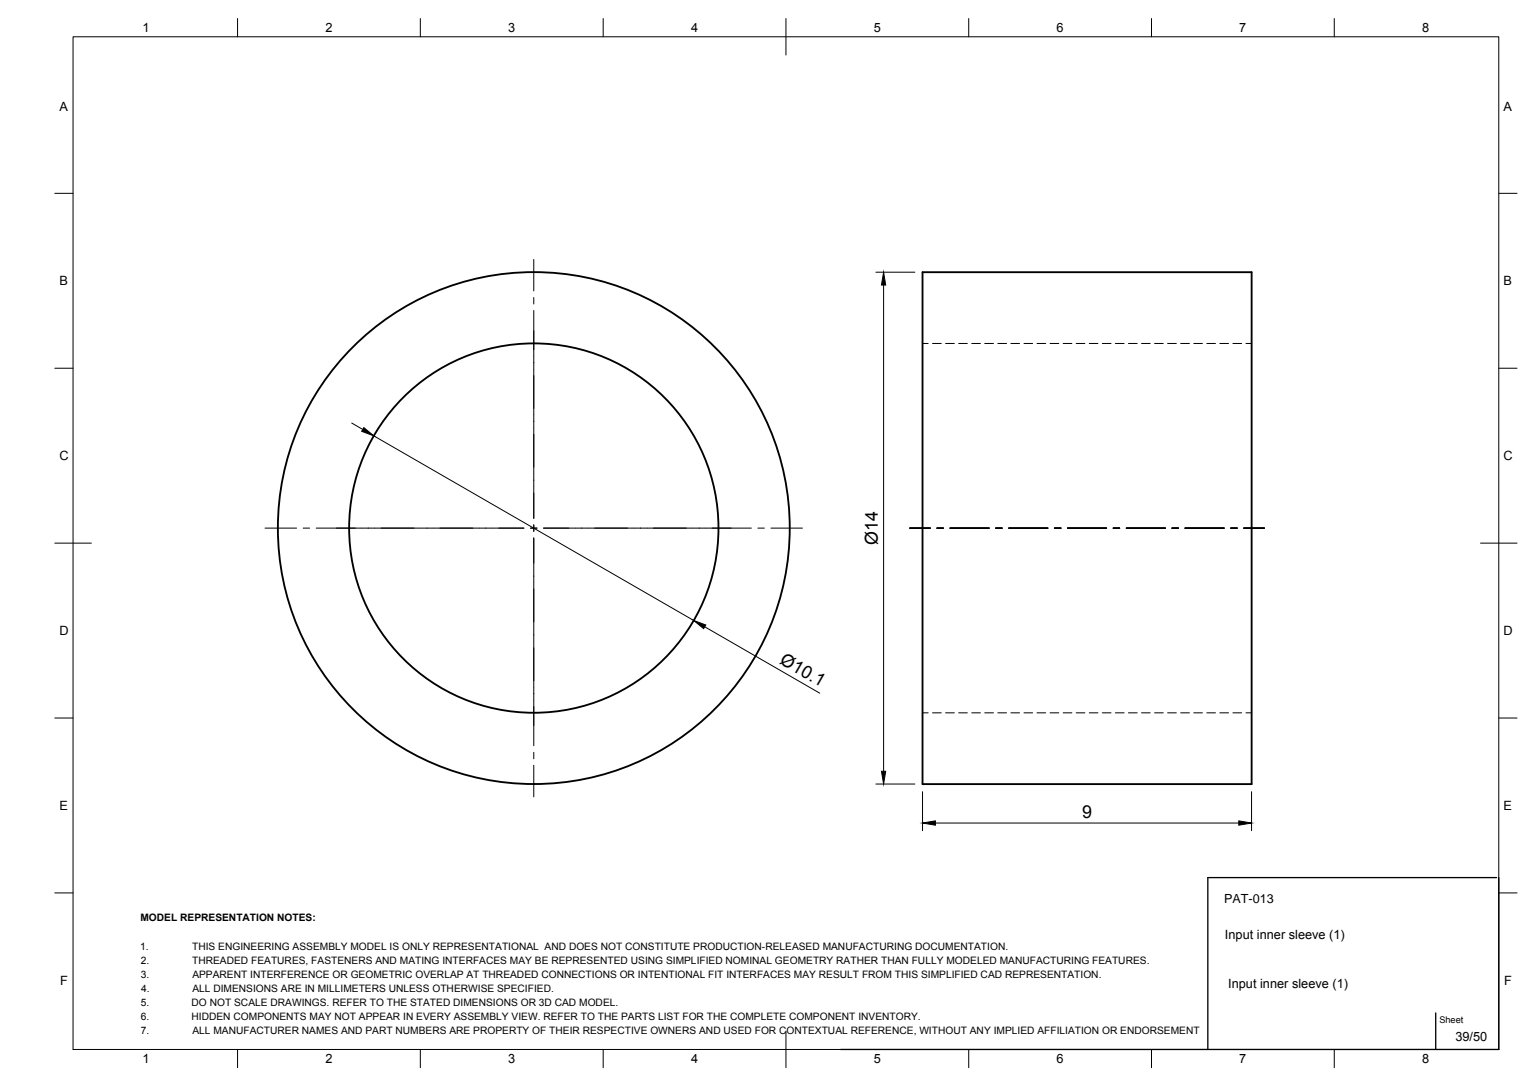
ISO-10303-21;
HEADER;
/* Generated by software containing ST-Developer
 * from STEP Tools, Inc. (www.steptools.com) 
 */

FILE_DESCRIPTION(
/* description */ ('Belt-driven linear axis on 2020 extrusion'),
/* implementation_level */ '2;1');

FILE_NAME(
/* name */ 'Input inner sleeve (1).step',
/* time_stamp */ '2026-10-28T03:26:09-07:00',
/* author */ (''),
/* organization */ (''),
/* preprocessor_version */ 'ST-DEVELOPER v20.2',
/* originating_system */ 'Autodesk Translation Framework v15.17.0.0',
/* authorisation */ '');

FILE_SCHEMA (('AUTOMOTIVE_DESIGN { 1 0 10303 214 3 1 1 }'));
ENDSEC;

DATA;
#10=MECHANICAL_DESIGN_GEOMETRIC_PRESENTATION_REPRESENTATION('',(#651),#20096);
#549=SHAPE_REPRESENTATION_RELATIONSHIP('SRR','None',#20348,#595);
#595=ADVANCED_BREP_SHAPE_REPRESENTATION('',(#706),#20079);
#651=STYLED_ITEM('',(#20636),#706);
#706=MANIFOLD_SOLID_BREP('Body1',#10965);
#847=FACE_BOUND('',#2420,.T.);
#848=FACE_BOUND('',#2422,.T.);
#1136=PLANE('',#12297);
#1137=PLANE('',#12298);
#1666=FACE_OUTER_BOUND('',#2417,.T.);
#1667=FACE_OUTER_BOUND('',#2418,.T.);
#1668=FACE_OUTER_BOUND('',#2419,.T.);
#1669=FACE_OUTER_BOUND('',#2421,.T.);
#2417=EDGE_LOOP('',(#9097,#9098,#9099,#9100));
#2418=EDGE_LOOP('',(#9101,#9102,#9103,#9104));
#2419=EDGE_LOOP('',(#9105));
#2420=EDGE_LOOP('',(#9106));
#2421=EDGE_LOOP('',(#9107));
#2422=EDGE_LOOP('',(#9108));
#3226=LINE('',#18577,#4083);
#3227=LINE('',#18583,#4084);
#4083=VECTOR('',#14952,0.505000000000003);
#4084=VECTOR('',#14959,0.700000000000003);
#4720=CIRCLE('',#12292,0.505000000000003);
#4721=CIRCLE('',#12293,0.505000000000003);
#4722=CIRCLE('',#12295,0.700000000000003);
#4723=CIRCLE('',#12296,0.700000000000003);
#5515=VERTEX_POINT('',#18574);
#5516=VERTEX_POINT('',#18576);
#5517=VERTEX_POINT('',#18580);
#5518=VERTEX_POINT('',#18582);
#6763=EDGE_CURVE('',#5515,#5515,#4720,.T.);
#6764=EDGE_CURVE('',#5515,#5516,#3226,.T.);
#6765=EDGE_CURVE('',#5516,#5516,#4721,.T.);
#6766=EDGE_CURVE('',#5517,#5517,#4722,.T.);
#6767=EDGE_CURVE('',#5517,#5518,#3227,.T.);
#6768=EDGE_CURVE('',#5518,#5518,#4723,.T.);
#9097=ORIENTED_EDGE('',*,*,#6763,.F.);
#9098=ORIENTED_EDGE('',*,*,#6764,.T.);
#9099=ORIENTED_EDGE('',*,*,#6765,.T.);
#9100=ORIENTED_EDGE('',*,*,#6764,.F.);
#9101=ORIENTED_EDGE('',*,*,#6766,.F.);
#9102=ORIENTED_EDGE('',*,*,#6767,.T.);
#9103=ORIENTED_EDGE('',*,*,#6768,.T.);
#9104=ORIENTED_EDGE('',*,*,#6767,.F.);
#9105=ORIENTED_EDGE('',*,*,#6766,.T.);
#9106=ORIENTED_EDGE('',*,*,#6763,.T.);
#9107=ORIENTED_EDGE('',*,*,#6768,.F.);
#9108=ORIENTED_EDGE('',*,*,#6765,.F.);
#10221=CYLINDRICAL_SURFACE('',#12291,0.505000000000003);
#10222=CYLINDRICAL_SURFACE('',#12294,0.700000000000003);
#10717=ADVANCED_FACE('',(#1666),#10221,.F.);
#10718=ADVANCED_FACE('',(#1667),#10222,.T.);
#10719=ADVANCED_FACE('',(#1668,#847),#1136,.T.);
#10720=ADVANCED_FACE('',(#1669,#848),#1137,.F.);
#10965=CLOSED_SHELL('',(#10717,#10718,#10719,#10720));
#12290=AXIS2_PLACEMENT_3D('',#18572,#14946,#14947);
#12291=AXIS2_PLACEMENT_3D('',#18573,#14948,#14949);
#12292=AXIS2_PLACEMENT_3D('',#18575,#14950,#14951);
#12293=AXIS2_PLACEMENT_3D('',#18578,#14953,#14954);
#12294=AXIS2_PLACEMENT_3D('',#18579,#14955,#14956);
#12295=AXIS2_PLACEMENT_3D('',#18581,#14957,#14958);
#12296=AXIS2_PLACEMENT_3D('',#18584,#14960,#14961);
#12297=AXIS2_PLACEMENT_3D('',#18585,#14962,#14963);
#12298=AXIS2_PLACEMENT_3D('',#18586,#14964,#14965);
#14946=DIRECTION('axis',(0.,0.,1.));
#14947=DIRECTION('refdir',(1.,0.,0.));
#14948=DIRECTION('center_axis',(0.,1.,0.));
#14949=DIRECTION('ref_axis',(1.,0.,0.));
#14950=DIRECTION('center_axis',(0.,-1.,0.));
#14951=DIRECTION('ref_axis',(1.,0.,0.));
#14952=DIRECTION('',(0.,-1.,0.));
#14953=DIRECTION('center_axis',(0.,-1.,0.));
#14954=DIRECTION('ref_axis',(1.,0.,0.));
#14955=DIRECTION('center_axis',(0.,1.,0.));
#14956=DIRECTION('ref_axis',(1.,0.,0.));
#14957=DIRECTION('center_axis',(0.,1.,0.));
#14958=DIRECTION('ref_axis',(1.,0.,0.));
#14959=DIRECTION('',(0.,-1.,0.));
#14960=DIRECTION('center_axis',(0.,1.,0.));
#14961=DIRECTION('ref_axis',(1.,0.,0.));
#14962=DIRECTION('center_axis',(0.,1.,0.));
#14963=DIRECTION('ref_axis',(1.,0.,0.));
#14964=DIRECTION('center_axis',(0.,1.,0.));
#14965=DIRECTION('ref_axis',(1.,0.,0.));
#18572=CARTESIAN_POINT('',(0.,0.,0.));
#18573=CARTESIAN_POINT('Origin',(32.,-0.45,7.));
#18574=CARTESIAN_POINT('',(31.495,0.45,7.));
#18575=CARTESIAN_POINT('Origin',(32.,0.45,7.));
#18576=CARTESIAN_POINT('',(31.495,-0.45,7.));
#18577=CARTESIAN_POINT('',(31.495,-0.45,7.));
#18578=CARTESIAN_POINT('Origin',(32.,-0.45,7.));
#18579=CARTESIAN_POINT('Origin',(32.,-0.45,7.));
#18580=CARTESIAN_POINT('',(31.3,0.45,7.));
#18581=CARTESIAN_POINT('Origin',(32.,0.45,7.));
#18582=CARTESIAN_POINT('',(31.3,-0.45,7.));
#18583=CARTESIAN_POINT('',(31.3,-0.45,7.));
#18584=CARTESIAN_POINT('Origin',(32.,-0.45,7.));
#18585=CARTESIAN_POINT('Origin',(32.,0.45,7.));
#18586=CARTESIAN_POINT('Origin',(32.,-0.45,7.));
#20025=UNCERTAINTY_MEASURE_WITH_UNIT(LENGTH_MEASURE(0.001),#20097,
'DISTANCE_ACCURACY_VALUE',
'Maximum model space distance between geometric entities at asserted c
onnectivities');
#20042=UNCERTAINTY_MEASURE_WITH_UNIT(LENGTH_MEASURE(0.001),#20097,
'DISTANCE_ACCURACY_VALUE',
'Maximum model space distance between geometric entities at asserted c
onnectivities');
#20079=(
GEOMETRIC_REPRESENTATION_CONTEXT(3)
GLOBAL_UNCERTAINTY_ASSIGNED_CONTEXT((#20025))
GLOBAL_UNIT_ASSIGNED_CONTEXT((#20097,#20099,#20100))
REPRESENTATION_CONTEXT('','3D')
);
#20096=(
GEOMETRIC_REPRESENTATION_CONTEXT(3)
GLOBAL_UNCERTAINTY_ASSIGNED_CONTEXT((#20042))
GLOBAL_UNIT_ASSIGNED_CONTEXT((#20097,#20099,#20100))
REPRESENTATION_CONTEXT('','3D')
);
#20097=(
LENGTH_UNIT()
NAMED_UNIT(*)
SI_UNIT(.CENTI.,.METRE.)
);
#20099=(
NAMED_UNIT(*)
PLANE_ANGLE_UNIT()
SI_UNIT($,.RADIAN.)
);
#20100=(
NAMED_UNIT(*)
SI_UNIT($,.STERADIAN.)
SOLID_ANGLE_UNIT()
);
#20137=SHAPE_DEFINITION_REPRESENTATION(#20195,#20348);
#20195=PRODUCT_DEFINITION_SHAPE('',$,#20402);
#20348=SHAPE_REPRESENTATION('',(#12290),#20079);
#20365=PRODUCT_DEFINITION_CONTEXT('part definition',#20526,'design');
#20402=PRODUCT_DEFINITION('Input inner sleeve (1)',
'Input inner sleeve (1)',#20455,#20365);
#20455=PRODUCT_DEFINITION_FORMATION('',$,#20564);
#20526=APPLICATION_CONTEXT(
'Core Data for Automotive Mechanical Design Process');
#20527=PRODUCT_CONTEXT('part definition',#20526,'mechanical');
#20564=PRODUCT('Input inner sleeve (1)','Input inner sleeve (1)',
'Input inner sleeve (1)',(#20527));
#20630=COLOUR_RGB('Light Blue',0.38,0.62,0.78);
#20631=FILL_AREA_STYLE_COLOUR('',#20630);
#20632=FILL_AREA_STYLE('',(#20631));
#20633=SURFACE_STYLE_FILL_AREA(#20632);
#20634=SURFACE_SIDE_STYLE('',(#20633));
#20635=SURFACE_STYLE_USAGE(.BOTH.,#20634);
#20636=PRESENTATION_STYLE_ASSIGNMENT((#20635));
ENDSEC;
END-ISO-10303-21;
